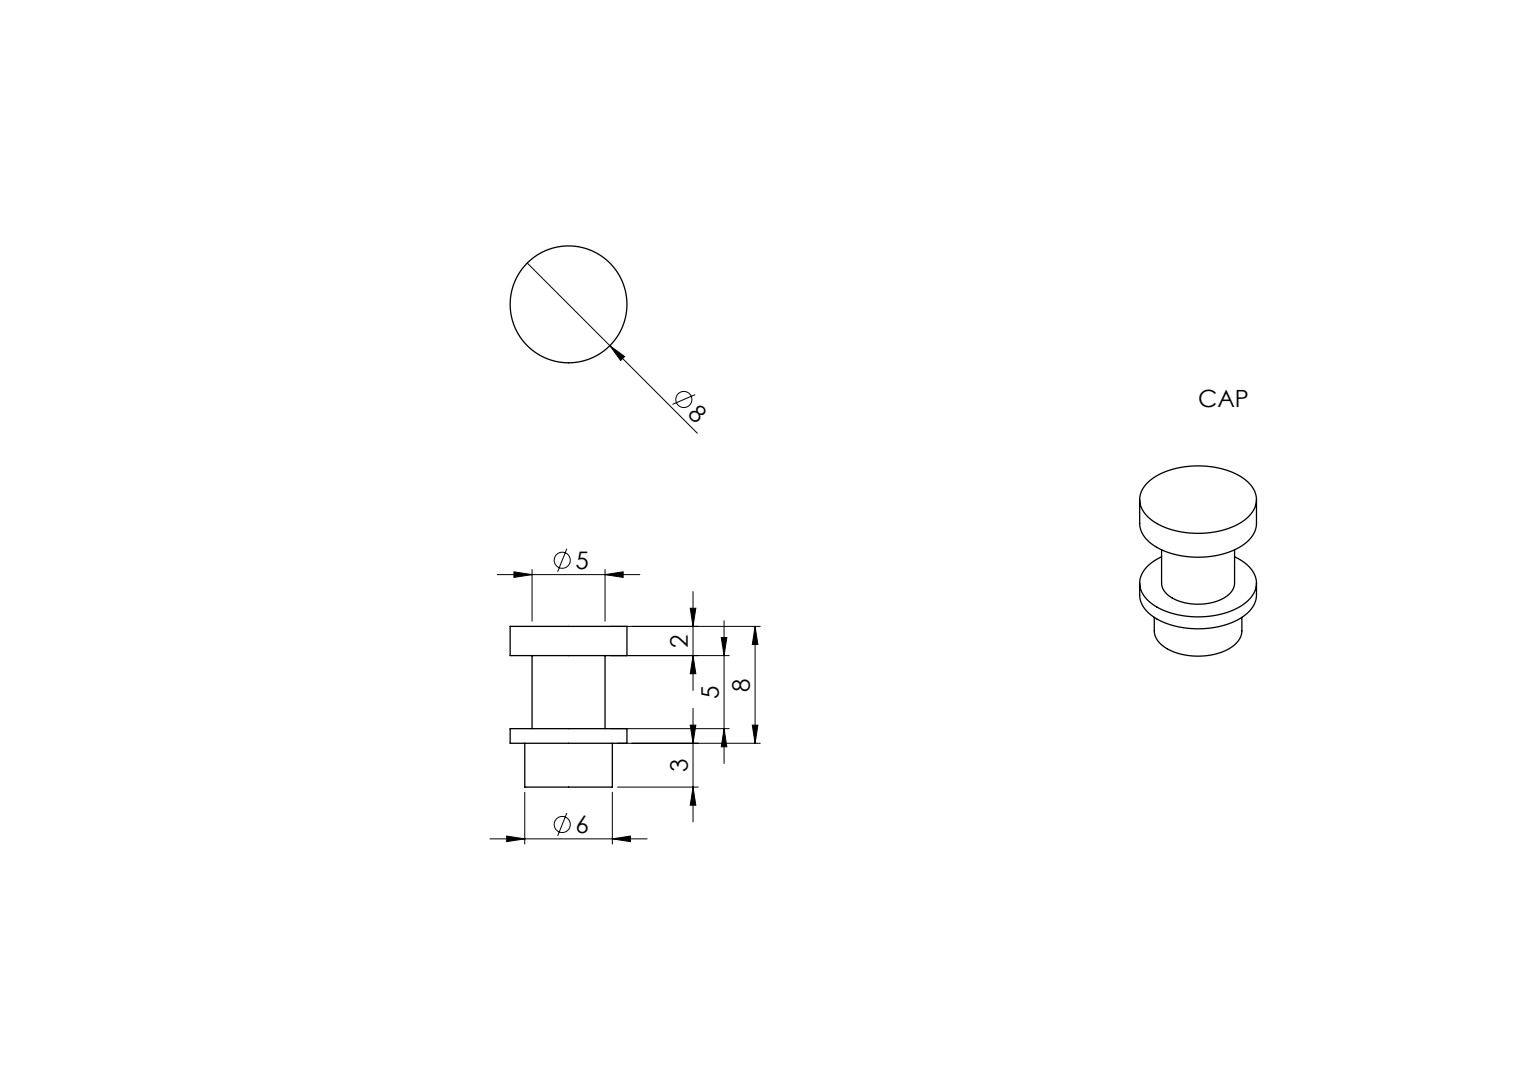
ISO-10303-21;
HEADER;
FILE_DESCRIPTION (('STEP AP214'),
    '1' );
FILE_NAME ('cap.step',
    '2026-10-27T10:49:47',
    ( '' ),
    ( '' ),
    'SwSTEP 2.0',
    'SolidWorks 2026',
    '' );
FILE_SCHEMA (( 'AUTOMOTIVE_DESIGN' ));
ENDSEC;

DATA;
#26=CARTESIAN_POINT ( 'NONE',  ( 4.898587196589412829E-16, 81.00000000000001421, 4.000000000000000000 ) ) ;
#47=( GEOMETRIC_REPRESENTATION_CONTEXT ( 3 ) GLOBAL_UNCERTAINTY_ASSIGNED_CONTEXT ( ( #2399 ) ) GLOBAL_UNIT_ASSIGNED_CONTEXT ( ( #4022, #5674, #2943 ) ) REPRESENTATION_CONTEXT ( 'NONE', 'WORKASPACE' ) );
#72=DIRECTION ( 'NONE',  ( -0.000000000000000000, 1.000000000000000000, -0.000000000000000000 ) ) ;
#89=LINE ( 'NONE', #7305, #4201 ) ;
#131=ADVANCED_FACE ( 'NONE', ( #1342 ), #6353, .T. ) ;
#147=AXIS2_PLACEMENT_3D ( 'NONE', #204, #847, #6661 ) ;
#150=FACE_OUTER_BOUND ( 'NONE', #5421, .T. ) ;
#154=VERTEX_POINT ( 'NONE', #6883 ) ;
#201=VECTOR ( 'NONE', #4183, 1000.000000000000000 ) ;
#204=CARTESIAN_POINT ( 'NONE',  ( 0.000000000000000000, 74.00000000000001421, 0.000000000000000000 ) ) ;
#268=FACE_OUTER_BOUND ( 'NONE', #8425, .T. ) ;
#292=AXIS2_PLACEMENT_3D ( 'NONE', #3378, #6815, #3894 ) ;
#297=DIRECTION ( 'NONE',  ( 0.000000000000000000, 0.000000000000000000, 1.000000000000000000 ) ) ;
#349=PRODUCT_DEFINITION ( 'UNKNOWN', '', #5751, #3204 ) ;
#350=DIRECTION ( 'NONE',  ( 0.000000000000000000, 1.000000000000000000, 0.000000000000000000 ) ) ;
#372=ORIENTED_EDGE ( 'NONE', *, *, #5983, .F. ) ;
#397=CYLINDRICAL_SURFACE ( 'NONE', #2530, 4.000000000000000000 ) ;
#400=EDGE_LOOP ( 'NONE', ( #2352, #922 ) ) ;
#408=ORIENTED_EDGE ( 'NONE', *, *, #9125, .F. ) ;
#409=( GEOMETRIC_REPRESENTATION_CONTEXT ( 3 ) GLOBAL_UNCERTAINTY_ASSIGNED_CONTEXT ( ( #1055 ) ) GLOBAL_UNIT_ASSIGNED_CONTEXT ( ( #5104, #7442, #1066 ) ) REPRESENTATION_CONTEXT ( 'NONE', 'WORKASPACE' ) );
#438=DIRECTION ( 'NONE',  ( -0.000000000000000000, -1.000000000000000000, -0.000000000000000000 ) ) ;
#443=CIRCLE ( 'NONE', #7579, 2.500000000000000000 ) ;
#455=VECTOR ( 'NONE', #7883, 1000.000000000000000 ) ;
#507=CARTESIAN_POINT ( 'NONE',  ( 4.898587196589412829E-16, 73.00000000000001421, 4.000000000000000000 ) ) ;
#537=DIRECTION ( 'NONE',  ( 0.000000000000000000, 0.000000000000000000, 1.000000000000000000 ) ) ;
#582=CARTESIAN_POINT ( 'NONE',  ( 0.000000000000000000, 74.00000000000001421, 2.500000000000000000 ) ) ;
#591=AXIS2_PLACEMENT_3D ( 'NONE', #8216, #7514, #537 ) ;
#594=FACE_OUTER_BOUND ( 'NONE', #5132, .T. ) ;
#612=CIRCLE ( 'NONE', #2974, 3.000000000000000444 ) ;
#624=DIRECTION ( 'NONE',  ( 0.000000000000000000, 0.000000000000000000, -1.000000000000000000 ) ) ;
#634=DIRECTION ( 'NONE',  ( -0.000000000000000000, -1.000000000000000000, -0.000000000000000000 ) ) ;
#641=DIRECTION ( 'NONE',  ( 0.000000000000000000, 1.000000000000000000, 0.000000000000000000 ) ) ;
#690=DIRECTION ( 'NONE',  ( 0.000000000000000000, 0.000000000000000000, 1.000000000000000000 ) ) ;
#691=PRODUCT ( 'cap', 'cap', '', ( #8871 ) ) ;
#724=AXIS2_PLACEMENT_3D ( 'NONE', #8229, #4642, #1153 ) ;
#847=DIRECTION ( 'NONE',  ( 0.000000000000000000, 1.000000000000000000, 0.000000000000000000 ) ) ;
#888=AXIS2_PLACEMENT_3D ( 'NONE', #4026, #9081, #6861 ) ;
#893=CARTESIAN_POINT ( 'NONE',  ( 0.000000000000000000, 79.00000000000001421, 0.000000000000000000 ) ) ;
#922=ORIENTED_EDGE ( 'NONE', *, *, #8343, .T. ) ;
#969=SURFACE_STYLE_USAGE ( .BOTH. , #8693 ) ;
#974=EDGE_LOOP ( 'NONE', ( #8366, #1071 ) ) ;
#989=FACE_BOUND ( 'NONE', #6645, .T. ) ;
#1041=CYLINDRICAL_SURFACE ( 'NONE', #7416, 3.000000000000000444 ) ;
#1048=ORIENTED_EDGE ( 'NONE', *, *, #8424, .T. ) ;
#1055=UNCERTAINTY_MEASURE_WITH_UNIT (LENGTH_MEASURE( 1.000000000000000082E-05 ), #5104, 'distance_accuracy_value', 'NONE');
#1066=( NAMED_UNIT ( * ) SI_UNIT ( $, .STERADIAN. ) SOLID_ANGLE_UNIT ( ) );
#1071=ORIENTED_EDGE ( 'NONE', *, *, #1671, .T. ) ;
#1106=ORIENTED_EDGE ( 'NONE', *, *, #6600, .F. ) ;
#1153=DIRECTION ( 'NONE',  ( 0.000000000000000000, 0.000000000000000000, 1.000000000000000000 ) ) ;
#1168=DIRECTION ( 'NONE',  ( 0.000000000000000000, 0.000000000000000000, 1.000000000000000000 ) ) ;
#1182=CIRCLE ( 'NONE', #724, 3.000000000000000444 ) ;
#1184=EDGE_CURVE ( 'NONE', #3304, #2164, #5654, .T. ) ;
#1191=CIRCLE ( 'NONE', #292, 2.500000000000000000 ) ;
#1216=ORIENTED_EDGE ( 'NONE', *, *, #4101, .T. ) ;
#1230=DIRECTION ( 'NONE',  ( 0.000000000000000000, 0.000000000000000000, 1.000000000000000000 ) ) ;
#1251=AXIS2_PLACEMENT_3D ( 'NONE', #3620, #641, #4139 ) ;
#1330=ORIENTED_EDGE ( 'NONE', *, *, #8424, .F. ) ;
#1333=DIRECTION ( 'NONE',  ( -0.000000000000000000, -1.000000000000000000, -0.000000000000000000 ) ) ;
#1342=FACE_OUTER_BOUND ( 'NONE', #5979, .T. ) ;
#1366=CARTESIAN_POINT ( 'NONE',  ( 0.000000000000000000, 74.00000000000001421, 0.000000000000000000 ) ) ;
#1367=DIRECTION ( 'NONE',  ( 0.000000000000000000, 1.000000000000000000, 0.000000000000000000 ) ) ;
#1372=CARTESIAN_POINT ( 'NONE',  ( 0.000000000000000000, 79.00000000000001421, -4.000000000000000000 ) ) ;
#1423=CARTESIAN_POINT ( 'NONE',  ( 4.898587196589412829E-16, 81.00000000000001421, 4.000000000000000000 ) ) ;
#1434=VERTEX_POINT ( 'NONE', #7055 ) ;
#1465=LINE ( 'NONE', #5884, #5657 ) ;
#1473=CARTESIAN_POINT ( 'NONE',  ( 0.000000000000000000, 81.00000000000001421, 0.000000000000000000 ) ) ;
#1539=CIRCLE ( 'NONE', #1251, 4.000000000000000000 ) ;
#1631=ORIENTED_EDGE ( 'NONE', *, *, #8037, .F. ) ;
#1635=AXIS2_PLACEMENT_3D ( 'NONE', #8434, #6111, #4845 ) ;
#1646=ORIENTED_EDGE ( 'NONE', *, *, #5983, .T. ) ;
#1651=ORIENTED_EDGE ( 'NONE', *, *, #2549, .T. ) ;
#1671=EDGE_CURVE ( 'NONE', #2249, #5349, #3580, .T. ) ;
#1719=PRESENTATION_STYLE_ASSIGNMENT (( #969 ) ) ;
#1822=VERTEX_POINT ( 'NONE', #8975 ) ;
#1853=ORIENTED_EDGE ( 'NONE', *, *, #2021, .F. ) ;
#1854=DIRECTION ( 'NONE',  ( -0.000000000000000000, -1.000000000000000000, -0.000000000000000000 ) ) ;
#1870=SHAPE_DEFINITION_REPRESENTATION ( #2935, #2791 ) ;
#1878=CARTESIAN_POINT ( 'NONE',  ( 0.000000000000000000, 70.00000000000000000, 0.000000000000000000 ) ) ;
#1886=DIRECTION ( 'NONE',  ( 0.000000000000000000, 1.000000000000000000, 0.000000000000000000 ) ) ;
#1892=FACE_OUTER_BOUND ( 'NONE', #5432, .T. ) ;
#1911=ORIENTED_EDGE ( 'NONE', *, *, #6017, .F. ) ;
#1985=ORIENTED_EDGE ( 'NONE', *, *, #8607, .F. ) ;
#2001=CARTESIAN_POINT ( 'NONE',  ( 0.000000000000000000, 81.00000000000001421, 0.000000000000000000 ) ) ;
#2018=EDGE_CURVE ( 'NONE', #3890, #7425, #4835, .T. ) ;
#2021=EDGE_CURVE ( 'NONE', #1822, #7425, #5506, .T. ) ;
#2075=AXIS2_PLACEMENT_3D ( 'NONE', #893, #5822, #7966 ) ;
#2095=AXIS2_PLACEMENT_3D ( 'NONE', #5123, #4435, #8712 ) ;
#2118=AXIS2_PLACEMENT_3D ( 'NONE', #2001, #7761, #2656 ) ;
#2125=DIRECTION ( 'NONE',  ( -0.000000000000000000, -1.000000000000000000, -0.000000000000000000 ) ) ;
#2132=LINE ( 'NONE', #2219, #201 ) ;
#2154=EDGE_CURVE ( 'NONE', #6474, #3890, #612, .T. ) ;
#2164=VERTEX_POINT ( 'NONE', #507 ) ;
#2219=CARTESIAN_POINT ( 'NONE',  ( 0.000000000000000000, 74.00000000000001421, 2.500000000000000000 ) ) ;
#2241=VECTOR ( 'NONE', #72, 1000.000000000000000 ) ;
#2249=VERTEX_POINT ( 'NONE', #9007 ) ;
#2274=CARTESIAN_POINT ( 'NONE',  ( 3.061616997868383141E-16, 79.00000000000001421, -2.500000000000000000 ) ) ;
#2304=EDGE_CURVE ( 'NONE', #6523, #3606, #2746, .T. ) ;
#2352=ORIENTED_EDGE ( 'NONE', *, *, #4698, .T. ) ;
#2392=CARTESIAN_POINT ( 'NONE',  ( 0.000000000000000000, 73.00000000000001421, -4.000000000000000000 ) ) ;
#2399=UNCERTAINTY_MEASURE_WITH_UNIT (LENGTH_MEASURE( 1.000000000000000082E-05 ), #4022, 'distance_accuracy_value', 'NONE');
#2447=FACE_OUTER_BOUND ( 'NONE', #4238, .T. ) ;
#2491=ORIENTED_EDGE ( 'NONE', *, *, #2832, .F. ) ;
#2530=AXIS2_PLACEMENT_3D ( 'NONE', #6216, #1854, #4589 ) ;
#2538=ADVANCED_BREP_SHAPE_REPRESENTATION ( '', ( #5399, #888 ), #7241 ) ;
#2539=CIRCLE ( 'NONE', #7592, 2.500000000000000000 ) ;
#2549=EDGE_CURVE ( 'NONE', #5349, #2876, #1465, .T. ) ;
#2574=ORIENTED_EDGE ( 'NONE', *, *, #3984, .F. ) ;
#2587=MECHANICAL_DESIGN_GEOMETRIC_PRESENTATION_REPRESENTATION('',(#8813),#47);
#2656=DIRECTION ( 'NONE',  ( 0.000000000000000000, 0.000000000000000000, -1.000000000000000000 ) ) ;
#2677=AXIS2_PLACEMENT_3D ( 'NONE', #8411, #634, #5035 ) ;
#2698=DIRECTION ( 'NONE',  ( 0.000000000000000000, 0.000000000000000000, 1.000000000000000000 ) ) ;
#2731=CIRCLE ( 'NONE', #2874, 2.500000000000000000 ) ;
#2746=LINE ( 'NONE', #7895, #2241 ) ;
#2782=ADVANCED_FACE ( 'NONE', ( #8360 ), #397, .T. ) ;
#2791=SHAPE_REPRESENTATION ( 'cap', ( #888 ), #7241 ) ;
#2832=EDGE_CURVE ( 'NONE', #154, #2876, #9188, .T. ) ;
#2874=AXIS2_PLACEMENT_3D ( 'NONE', #6008, #1886, #6200 ) ;
#2876=VERTEX_POINT ( 'NONE', #1372 ) ;
#2907=CYLINDRICAL_SURFACE ( 'NONE', #7179, 2.500000000000000000 ) ;
#2909=FACE_OUTER_BOUND ( 'NONE', #4484, .T. ) ;
#2935=PRODUCT_DEFINITION_SHAPE ( 'NONE', 'NONE',  #349 ) ;
#2943=( NAMED_UNIT ( * ) SI_UNIT ( $, .STERADIAN. ) SOLID_ANGLE_UNIT ( ) );
#2952=DIRECTION ( 'NONE',  ( 0.000000000000000000, 1.000000000000000000, 0.000000000000000000 ) ) ;
#2974=AXIS2_PLACEMENT_3D ( 'NONE', #8866, #9054, #2698 ) ;
#2977=CIRCLE ( 'NONE', #3717, 3.000000000000000444 ) ;
#2998=CARTESIAN_POINT ( 'NONE',  ( 3.673940397442060361E-16, 73.00000000000001421, 3.000000000000000444 ) ) ;
#3039=DIRECTION ( 'NONE',  ( -0.000000000000000000, -1.000000000000000000, -0.000000000000000000 ) ) ;
#3043=CIRCLE ( 'NONE', #8238, 4.000000000000000000 ) ;
#3047=CARTESIAN_POINT ( 'NONE',  ( 0.000000000000000000, 73.00000000000001421, 0.000000000000000000 ) ) ;
#3055=PLANE ( 'NONE',  #147 ) ;
#3077=FILL_AREA_STYLE ('',( #8043 ) ) ;
#3084=EDGE_LOOP ( 'NONE', ( #7913, #1646 ) ) ;
#3121=PLANE ( 'NONE',  #1635 ) ;
#3133=AXIS2_PLACEMENT_3D ( 'NONE', #3047, #3741, #8659 ) ;
#3135=EDGE_CURVE ( 'NONE', #6474, #1822, #5027, .T. ) ;
#3155=ORIENTED_EDGE ( 'NONE', *, *, #1671, .F. ) ;
#3163=ADVANCED_FACE ( 'NONE', ( #989, #5222 ), #3055, .T. ) ;
#3167=CARTESIAN_POINT ( 'NONE',  ( 0.000000000000000000, 74.00000000000001421, 0.000000000000000000 ) ) ;
#3204=PRODUCT_DEFINITION_CONTEXT ( 'detailed design', #5531, 'design' ) ;
#3205=VERTEX_POINT ( 'NONE', #2392 ) ;
#3237=CYLINDRICAL_SURFACE ( 'NONE', #7792, 4.000000000000000000 ) ;
#3256=ORIENTED_EDGE ( 'NONE', *, *, #3453, .T. ) ;
#3288=DIRECTION ( 'NONE',  ( 0.000000000000000000, 0.000000000000000000, 1.000000000000000000 ) ) ;
#3304=VERTEX_POINT ( 'NONE', #6759 ) ;
#3314=DIRECTION ( 'NONE',  ( -0.000000000000000000, -1.000000000000000000, -0.000000000000000000 ) ) ;
#3321=ORIENTED_EDGE ( 'NONE', *, *, #8037, .T. ) ;
#3378=CARTESIAN_POINT ( 'NONE',  ( 0.000000000000000000, 79.00000000000001421, 0.000000000000000000 ) ) ;
#3453=EDGE_CURVE ( 'NONE', #4194, #6523, #2539, .T. ) ;
#3580=CIRCLE ( 'NONE', #2095, 4.000000000000000000 ) ;
#3606=VERTEX_POINT ( 'NONE', #2274 ) ;
#3620=CARTESIAN_POINT ( 'NONE',  ( 0.000000000000000000, 74.00000000000001421, 0.000000000000000000 ) ) ;
#3643=CARTESIAN_POINT ( 'NONE',  ( 0.000000000000000000, 70.00000000000000000, 0.000000000000000000 ) ) ;
#3655=ORIENTED_EDGE ( 'NONE', *, *, #8343, .F. ) ;
#3717=AXIS2_PLACEMENT_3D ( 'NONE', #4887, #4762, #1230 ) ;
#3741=DIRECTION ( 'NONE',  ( 0.000000000000000000, 1.000000000000000000, 0.000000000000000000 ) ) ;
#3743=FACE_OUTER_BOUND ( 'NONE', #6302, .T. ) ;
#3772=SURFACE_STYLE_FILL_AREA ( #3077 ) ;
#3777=ORIENTED_EDGE ( 'NONE', *, *, #9125, .T. ) ;
#3794=CARTESIAN_POINT ( 'NONE',  ( 0.000000000000000000, 73.00000000000001421, -3.000000000000000444 ) ) ;
#3847=DIRECTION ( 'NONE',  ( -0.000000000000000000, -1.000000000000000000, -0.000000000000000000 ) ) ;
#3868=CIRCLE ( 'NONE', #5934, 4.000000000000000000 ) ;
#3890=VERTEX_POINT ( 'NONE', #2998 ) ;
#3894=DIRECTION ( 'NONE',  ( 0.000000000000000000, 0.000000000000000000, 1.000000000000000000 ) ) ;
#3900=ORIENTED_EDGE ( 'NONE', *, *, #1184, .T. ) ;
#3903=CARTESIAN_POINT ( 'NONE',  ( 3.673940397442060361E-16, 70.00000000000000000, 3.000000000000000444 ) ) ;
#3935=CARTESIAN_POINT ( 'NONE',  ( 0.000000000000000000, 73.00000000000001421, -3.000000000000000444 ) ) ;
#3984=EDGE_CURVE ( 'NONE', #2164, #3205, #7138, .T. ) ;
#4022=( LENGTH_UNIT ( ) NAMED_UNIT ( * ) SI_UNIT ( .MILLI., .METRE. ) );
#4026=CARTESIAN_POINT ( 'NONE',  ( 0.000000000000000000, 0.000000000000000000, 0.000000000000000000 ) ) ;
#4101=EDGE_CURVE ( 'NONE', #5172, #3205, #89, .T. ) ;
#4118=DIRECTION ( 'NONE',  ( -0.000000000000000000, -1.000000000000000000, -0.000000000000000000 ) ) ;
#4139=DIRECTION ( 'NONE',  ( 0.000000000000000000, 0.000000000000000000, 1.000000000000000000 ) ) ;
#4183=DIRECTION ( 'NONE',  ( -0.000000000000000000, 1.000000000000000000, -0.000000000000000000 ) ) ;
#4194=VERTEX_POINT ( 'NONE', #582 ) ;
#4201=VECTOR ( 'NONE', #3039, 1000.000000000000000 ) ;
#4238=EDGE_LOOP ( 'NONE', ( #1631, #1106, #1651, #5055 ) ) ;
#4275=ADVANCED_FACE ( 'NONE', ( #2909 ), #5683, .T. ) ;
#4316=DIRECTION ( 'NONE',  ( 0.000000000000000000, 1.000000000000000000, 0.000000000000000000 ) ) ;
#4349=EDGE_LOOP ( 'NONE', ( #6694, #6748 ) ) ;
#4435=DIRECTION ( 'NONE',  ( 0.000000000000000000, 1.000000000000000000, 0.000000000000000000 ) ) ;
#4466=ORIENTED_EDGE ( 'NONE', *, *, #3453, .F. ) ;
#4484=EDGE_LOOP ( 'NONE', ( #6407, #6798, #7135, #4561 ) ) ;
#4561=ORIENTED_EDGE ( 'NONE', *, *, #2021, .T. ) ;
#4589=DIRECTION ( 'NONE',  ( 0.000000000000000000, 0.000000000000000000, -1.000000000000000000 ) ) ;
#4592=ORIENTED_EDGE ( 'NONE', *, *, #2304, .F. ) ;
#4627=DIRECTION ( 'NONE',  ( 0.000000000000000000, 0.000000000000000000, -1.000000000000000000 ) ) ;
#4631=DIRECTION ( 'NONE',  ( 0.000000000000000000, 1.000000000000000000, 0.000000000000000000 ) ) ;
#4642=DIRECTION ( 'NONE',  ( 0.000000000000000000, 1.000000000000000000, 0.000000000000000000 ) ) ;
#4674=DIRECTION ( 'NONE',  ( -0.000000000000000000, -1.000000000000000000, -0.000000000000000000 ) ) ;
#4698=EDGE_CURVE ( 'NONE', #1434, #3606, #2731, .T. ) ;
#4762=DIRECTION ( 'NONE',  ( 0.000000000000000000, 1.000000000000000000, 0.000000000000000000 ) ) ;
#4835=LINE ( 'NONE', #8244, #7738 ) ;
#4845=DIRECTION ( 'NONE',  ( 0.000000000000000000, -0.000000000000000000, 1.000000000000000000 ) ) ;
#4887=CARTESIAN_POINT ( 'NONE',  ( 0.000000000000000000, 70.00000000000000000, 0.000000000000000000 ) ) ;
#4892=DIRECTION ( 'NONE',  ( -0.000000000000000000, 1.000000000000000000, -0.000000000000000000 ) ) ;
#4962=CARTESIAN_POINT ( 'NONE',  ( 0.000000000000000000, 74.00000000000001421, 0.000000000000000000 ) ) ;
#4995=FACE_OUTER_BOUND ( 'NONE', #974, .T. ) ;
#5010=EDGE_LOOP ( 'NONE', ( #4592, #8857, #9090, #3655 ) ) ;
#5016=ADVANCED_FACE ( 'NONE', ( #5638 ), #2907, .T. ) ;
#5027=LINE ( 'NONE', #3794, #455 ) ;
#5035=DIRECTION ( 'NONE',  ( 0.000000000000000000, 0.000000000000000000, -1.000000000000000000 ) ) ;
#5053=DIRECTION ( 'NONE',  ( 0.000000000000000000, 1.000000000000000000, 0.000000000000000000 ) ) ;
#5055=ORIENTED_EDGE ( 'NONE', *, *, #8607, .T. ) ;
#5104=( LENGTH_UNIT ( ) NAMED_UNIT ( * ) SI_UNIT ( .MILLI., .METRE. ) );
#5110=ORIENTED_EDGE ( 'NONE', *, *, #4698, .F. ) ;
#5123=CARTESIAN_POINT ( 'NONE',  ( 0.000000000000000000, 81.00000000000001421, 0.000000000000000000 ) ) ;
#5132=EDGE_LOOP ( 'NONE', ( #372, #3900, #8266, #7731 ) ) ;
#5172=VERTEX_POINT ( 'NONE', #7412 ) ;
#5222=FACE_OUTER_BOUND ( 'NONE', #3084, .T. ) ;
#5314=DIRECTION ( 'NONE',  ( 0.000000000000000000, 1.000000000000000000, 0.000000000000000000 ) ) ;
#5349=VERTEX_POINT ( 'NONE', #5358 ) ;
#5358=CARTESIAN_POINT ( 'NONE',  ( 0.000000000000000000, 81.00000000000001421, -4.000000000000000000 ) ) ;
#5399=MANIFOLD_SOLID_BREP ( 'Cut-Extrude-Thin1', #6088 ) ;
#5421=EDGE_LOOP ( 'NONE', ( #1985, #2491 ) ) ;
#5432=EDGE_LOOP ( 'NONE', ( #8598, #6476, #3777, #8148 ) ) ;
#5506=CIRCLE ( 'NONE', #6100, 3.000000000000000444 ) ;
#5531=APPLICATION_CONTEXT ( 'automotive_design' ) ;
#5608=COLOUR_RGB ( '',0.8941176470588234615, 0.8941176470588234615, 0.8941176470588234615 ) ;
#5638=FACE_OUTER_BOUND ( 'NONE', #5010, .T. ) ;
#5654=LINE ( 'NONE', #1423, #6148 ) ;
#5657=VECTOR ( 'NONE', #3847, 1000.000000000000000 ) ;
#5674=( NAMED_UNIT ( * ) PLANE_ANGLE_UNIT ( ) SI_UNIT ( $, .RADIAN. ) );
#5683=CYLINDRICAL_SURFACE ( 'NONE', #7768, 3.000000000000000444 ) ;
#5751=PRODUCT_DEFINITION_FORMATION_WITH_SPECIFIED_SOURCE ( 'ANY', '', #691, .NOT_KNOWN. ) ;
#5782=AXIS2_PLACEMENT_3D ( 'NONE', #7174, #6466, #8059 ) ;
#5787=EDGE_LOOP ( 'NONE', ( #6426, #7090, #1216, #1048 ) ) ;
#5822=DIRECTION ( 'NONE',  ( 0.000000000000000000, 1.000000000000000000, 0.000000000000000000 ) ) ;
#5884=CARTESIAN_POINT ( 'NONE',  ( 0.000000000000000000, 81.00000000000001421, -4.000000000000000000 ) ) ;
#5914=PLANE ( 'NONE',  #7123 ) ;
#5934=AXIS2_PLACEMENT_3D ( 'NONE', #8855, #4631, #3288 ) ;
#5979=EDGE_LOOP ( 'NONE', ( #3155, #3321, #6412, #7752 ) ) ;
#5983=EDGE_CURVE ( 'NONE', #3304, #5172, #1539, .T. ) ;
#6008=CARTESIAN_POINT ( 'NONE',  ( 0.000000000000000000, 79.00000000000001421, 0.000000000000000000 ) ) ;
#6017=EDGE_CURVE ( 'NONE', #4194, #1434, #2132, .T. ) ;
#6061=CARTESIAN_POINT ( 'NONE',  ( 3.061616997868383141E-16, 74.00000000000001421, -2.500000000000000000 ) ) ;
#6068=CARTESIAN_POINT ( 'NONE',  ( 0.000000000000000000, 79.00000000000001421, 0.000000000000000000 ) ) ;
#6084=ADVANCED_FACE ( 'NONE', ( #4995 ), #6400, .T. ) ;
#6088=CLOSED_SHELL ( 'NONE', ( #131, #8881, #6622, #7934, #2782, #4275, #8600, #9033, #3163, #8563, #5016, #6084, #6475 ) ) ;
#6100=AXIS2_PLACEMENT_3D ( 'NONE', #1878, #7541, #1168 ) ;
#6111=DIRECTION ( 'NONE',  ( 0.000000000000000000, 1.000000000000000000, 0.000000000000000000 ) ) ;
#6148=VECTOR ( 'NONE', #2125, 1000.000000000000000 ) ;
#6163=CARTESIAN_POINT ( 'NONE',  ( 0.000000000000000000, 73.00000000000001421, 0.000000000000000000 ) ) ;
#6200=DIRECTION ( 'NONE',  ( 0.000000000000000000, 0.000000000000000000, 1.000000000000000000 ) ) ;
#6216=CARTESIAN_POINT ( 'NONE',  ( 0.000000000000000000, 81.00000000000001421, 0.000000000000000000 ) ) ;
#6302=EDGE_LOOP ( 'NONE', ( #1853, #408 ) ) ;
#6321=EDGE_LOOP ( 'NONE', ( #3256, #9044, #5110, #1911 ) ) ;
#6353=CYLINDRICAL_SURFACE ( 'NONE', #2118, 4.000000000000000000 ) ;
#6400=PLANE ( 'NONE',  #8231 ) ;
#6407=ORIENTED_EDGE ( 'NONE', *, *, #2018, .F. ) ;
#6412=ORIENTED_EDGE ( 'NONE', *, *, #2832, .T. ) ;
#6426=ORIENTED_EDGE ( 'NONE', *, *, #1184, .F. ) ;
#6444=DIRECTION ( 'NONE',  ( 0.000000000000000000, -0.000000000000000000, 1.000000000000000000 ) ) ;
#6466=DIRECTION ( 'NONE',  ( 0.000000000000000000, 1.000000000000000000, 0.000000000000000000 ) ) ;
#6474=VERTEX_POINT ( 'NONE', #3935 ) ;
#6475=ADVANCED_FACE ( 'NONE', ( #2447 ), #3237, .T. ) ;
#6476=ORIENTED_EDGE ( 'NONE', *, *, #2018, .T. ) ;
#6513=DIRECTION ( 'NONE',  ( 0.000000000000000000, -0.000000000000000000, 1.000000000000000000 ) ) ;
#6523=VERTEX_POINT ( 'NONE', #6061 ) ;
#6600=EDGE_CURVE ( 'NONE', #5349, #2249, #3043, .T. ) ;
#6622=ADVANCED_FACE ( 'NONE', ( #1892 ), #1041, .T. ) ;
#6639=FACE_BOUND ( 'NONE', #4349, .T. ) ;
#6645=EDGE_LOOP ( 'NONE', ( #4466, #8198 ) ) ;
#6661=DIRECTION ( 'NONE',  ( 0.000000000000000000, -0.000000000000000000, 1.000000000000000000 ) ) ;
#6694=ORIENTED_EDGE ( 'NONE', *, *, #2154, .T. ) ;
#6748=ORIENTED_EDGE ( 'NONE', *, *, #7785, .T. ) ;
#6759=CARTESIAN_POINT ( 'NONE',  ( 4.898587196589412829E-16, 74.00000000000001421, 4.000000000000000000 ) ) ;
#6798=ORIENTED_EDGE ( 'NONE', *, *, #2154, .F. ) ;
#6804=MECHANICAL_DESIGN_GEOMETRIC_PRESENTATION_REPRESENTATION('',(#7692),#409);
#6815=DIRECTION ( 'NONE',  ( 0.000000000000000000, 1.000000000000000000, 0.000000000000000000 ) ) ;
#6832=CIRCLE ( 'NONE', #5782, 4.000000000000000000 ) ;
#6861=DIRECTION ( 'NONE',  ( 1.000000000000000000, 0.000000000000000000, 0.000000000000000000 ) ) ;
#6883=CARTESIAN_POINT ( 'NONE',  ( 4.898587196589412829E-16, 79.00000000000001421, 4.000000000000000000 ) ) ;
#6997=DIRECTION ( 'NONE',  ( 0.000000000000000000, 0.000000000000000000, 1.000000000000000000 ) ) ;
#7055=CARTESIAN_POINT ( 'NONE',  ( 0.000000000000000000, 79.00000000000001421, 2.500000000000000000 ) ) ;
#7090=ORIENTED_EDGE ( 'NONE', *, *, #8447, .F. ) ;
#7123=AXIS2_PLACEMENT_3D ( 'NONE', #3643, #2952, #6513 ) ;
#7135=ORIENTED_EDGE ( 'NONE', *, *, #3135, .T. ) ;
#7138=CIRCLE ( 'NONE', #3133, 4.000000000000000000 ) ;
#7173=DIRECTION ( 'NONE',  ( 0.000000000000000000, 0.000000000000000000, 1.000000000000000000 ) ) ;
#7174=CARTESIAN_POINT ( 'NONE',  ( 0.000000000000000000, 79.00000000000001421, 0.000000000000000000 ) ) ;
#7179=AXIS2_PLACEMENT_3D ( 'NONE', #1366, #4892, #7173 ) ;
#7241=( GEOMETRIC_REPRESENTATION_CONTEXT ( 3 ) GLOBAL_UNCERTAINTY_ASSIGNED_CONTEXT ( ( #7475 ) ) GLOBAL_UNIT_ASSIGNED_CONTEXT ( ( #7774, #9155, #8426 ) ) REPRESENTATION_CONTEXT ( 'NONE', 'WORKASPACE' ) );
#7247=FACE_OUTER_BOUND ( 'NONE', #6321, .T. ) ;
#7305=CARTESIAN_POINT ( 'NONE',  ( 0.000000000000000000, 81.00000000000001421, -4.000000000000000000 ) ) ;
#7412=CARTESIAN_POINT ( 'NONE',  ( 0.000000000000000000, 74.00000000000001421, -4.000000000000000000 ) ) ;
#7416=AXIS2_PLACEMENT_3D ( 'NONE', #6163, #4674, #8167 ) ;
#7419=CARTESIAN_POINT ( 'NONE',  ( 0.000000000000000000, 81.00000000000001421, 0.000000000000000000 ) ) ;
#7425=VERTEX_POINT ( 'NONE', #3903 ) ;
#7442=( NAMED_UNIT ( * ) PLANE_ANGLE_UNIT ( ) SI_UNIT ( $, .RADIAN. ) );
#7475=UNCERTAINTY_MEASURE_WITH_UNIT (LENGTH_MEASURE( 1.000000000000000082E-05 ), #7774, 'distance_accuracy_value', 'NONE');
#7514=DIRECTION ( 'NONE',  ( 0.000000000000000000, 1.000000000000000000, 0.000000000000000000 ) ) ;
#7541=DIRECTION ( 'NONE',  ( 0.000000000000000000, 1.000000000000000000, 0.000000000000000000 ) ) ;
#7579=AXIS2_PLACEMENT_3D ( 'NONE', #7744, #1367, #6997 ) ;
#7583=AXIS2_PLACEMENT_3D ( 'NONE', #6068, #350, #8904 ) ;
#7592=AXIS2_PLACEMENT_3D ( 'NONE', #4962, #5053, #690 ) ;
#7692=STYLED_ITEM ( 'NONE', ( #1719 ), #2538 ) ;
#7708=LINE ( 'NONE', #26, #9049 ) ;
#7723=CIRCLE ( 'NONE', #591, 4.000000000000000000 ) ;
#7731=ORIENTED_EDGE ( 'NONE', *, *, #4101, .F. ) ;
#7738=VECTOR ( 'NONE', #3314, 1000.000000000000000 ) ;
#7744=CARTESIAN_POINT ( 'NONE',  ( 0.000000000000000000, 74.00000000000001421, 0.000000000000000000 ) ) ;
#7752=ORIENTED_EDGE ( 'NONE', *, *, #2549, .F. ) ;
#7761=DIRECTION ( 'NONE',  ( -0.000000000000000000, -1.000000000000000000, -0.000000000000000000 ) ) ;
#7768=AXIS2_PLACEMENT_3D ( 'NONE', #8440, #4118, #624 ) ;
#7774=( LENGTH_UNIT ( ) NAMED_UNIT ( * ) SI_UNIT ( .MILLI., .METRE. ) );
#7785=EDGE_CURVE ( 'NONE', #3890, #6474, #1182, .T. ) ;
#7792=AXIS2_PLACEMENT_3D ( 'NONE', #7419, #438, #4627 ) ;
#7883=DIRECTION ( 'NONE',  ( -0.000000000000000000, -1.000000000000000000, -0.000000000000000000 ) ) ;
#7895=CARTESIAN_POINT ( 'NONE',  ( 3.061616997868383141E-16, 74.00000000000001421, -2.500000000000000000 ) ) ;
#7913=ORIENTED_EDGE ( 'NONE', *, *, #8447, .T. ) ;
#7934=ADVANCED_FACE ( 'NONE', ( #594 ), #9142, .T. ) ;
#7951=CYLINDRICAL_SURFACE ( 'NONE', #8171, 2.500000000000000000 ) ;
#7965=APPLICATION_CONTEXT ( 'automotive_design' ) ;
#7966=DIRECTION ( 'NONE',  ( 0.000000000000000000, -0.000000000000000000, 1.000000000000000000 ) ) ;
#8010=PLANE ( 'NONE',  #2075 ) ;
#8037=EDGE_CURVE ( 'NONE', #2249, #154, #7708, .T. ) ;
#8042=DIRECTION ( 'NONE',  ( -0.000000000000000000, 1.000000000000000000, -0.000000000000000000 ) ) ;
#8043=FILL_AREA_STYLE_COLOUR ( '', #5608 ) ;
#8059=DIRECTION ( 'NONE',  ( 0.000000000000000000, 0.000000000000000000, 1.000000000000000000 ) ) ;
#8148=ORIENTED_EDGE ( 'NONE', *, *, #3135, .F. ) ;
#8167=DIRECTION ( 'NONE',  ( 0.000000000000000000, 0.000000000000000000, -1.000000000000000000 ) ) ;
#8171=AXIS2_PLACEMENT_3D ( 'NONE', #3167, #8042, #8785 ) ;
#8198=ORIENTED_EDGE ( 'NONE', *, *, #8471, .F. ) ;
#8216=CARTESIAN_POINT ( 'NONE',  ( 0.000000000000000000, 73.00000000000001421, 0.000000000000000000 ) ) ;
#8229=CARTESIAN_POINT ( 'NONE',  ( 0.000000000000000000, 73.00000000000001421, 0.000000000000000000 ) ) ;
#8231=AXIS2_PLACEMENT_3D ( 'NONE', #1473, #4316, #6444 ) ;
#8238=AXIS2_PLACEMENT_3D ( 'NONE', #8989, #5314, #297 ) ;
#8244=CARTESIAN_POINT ( 'NONE',  ( 3.673940397442060361E-16, 73.00000000000001421, 3.000000000000000444 ) ) ;
#8266=ORIENTED_EDGE ( 'NONE', *, *, #3984, .T. ) ;
#8343=EDGE_CURVE ( 'NONE', #3606, #1434, #1191, .T. ) ;
#8360=FACE_OUTER_BOUND ( 'NONE', #5787, .T. ) ;
#8366=ORIENTED_EDGE ( 'NONE', *, *, #6600, .T. ) ;
#8411=CARTESIAN_POINT ( 'NONE',  ( 0.000000000000000000, 81.00000000000001421, 0.000000000000000000 ) ) ;
#8424=EDGE_CURVE ( 'NONE', #3205, #2164, #7723, .T. ) ;
#8425=EDGE_LOOP ( 'NONE', ( #1330, #2574 ) ) ;
#8426=( NAMED_UNIT ( * ) SI_UNIT ( $, .STERADIAN. ) SOLID_ANGLE_UNIT ( ) );
#8434=CARTESIAN_POINT ( 'NONE',  ( 0.000000000000000000, 73.00000000000001421, 0.000000000000000000 ) ) ;
#8440=CARTESIAN_POINT ( 'NONE',  ( 0.000000000000000000, 73.00000000000001421, 0.000000000000000000 ) ) ;
#8447=EDGE_CURVE ( 'NONE', #5172, #3304, #3868, .T. ) ;
#8471=EDGE_CURVE ( 'NONE', #6523, #4194, #443, .T. ) ;
#8563=ADVANCED_FACE ( 'NONE', ( #8569, #150 ), #8010, .F. ) ;
#8569=FACE_BOUND ( 'NONE', #400, .T. ) ;
#8598=ORIENTED_EDGE ( 'NONE', *, *, #7785, .F. ) ;
#8600=ADVANCED_FACE ( 'NONE', ( #3743 ), #5914, .F. ) ;
#8607=EDGE_CURVE ( 'NONE', #2876, #154, #6832, .T. ) ;
#8659=DIRECTION ( 'NONE',  ( 0.000000000000000000, 0.000000000000000000, 1.000000000000000000 ) ) ;
#8693=SURFACE_SIDE_STYLE ('',( #3772 ) ) ;
#8712=DIRECTION ( 'NONE',  ( 0.000000000000000000, 0.000000000000000000, 1.000000000000000000 ) ) ;
#8738=SHAPE_REPRESENTATION_RELATIONSHIP ( 'NONE' , 'NONE' ,  #2791, #2538 ) ;
#8785=DIRECTION ( 'NONE',  ( 0.000000000000000000, 0.000000000000000000, 1.000000000000000000 ) ) ;
#8813=STYLED_ITEM('',(#9218),#5399);
#8855=CARTESIAN_POINT ( 'NONE',  ( 0.000000000000000000, 74.00000000000001421, 0.000000000000000000 ) ) ;
#8857=ORIENTED_EDGE ( 'NONE', *, *, #8471, .T. ) ;
#8866=CARTESIAN_POINT ( 'NONE',  ( 0.000000000000000000, 73.00000000000001421, 0.000000000000000000 ) ) ;
#8871=PRODUCT_CONTEXT ( 'NONE', #7965, 'mechanical' ) ;
#8881=ADVANCED_FACE ( 'NONE', ( #7247 ), #7951, .T. ) ;
#8904=DIRECTION ( 'NONE',  ( 0.000000000000000000, 0.000000000000000000, 1.000000000000000000 ) ) ;
#8975=CARTESIAN_POINT ( 'NONE',  ( 0.000000000000000000, 70.00000000000000000, -3.000000000000000444 ) ) ;
#8989=CARTESIAN_POINT ( 'NONE',  ( 0.000000000000000000, 81.00000000000001421, 0.000000000000000000 ) ) ;
#9007=CARTESIAN_POINT ( 'NONE',  ( 4.898587196589412829E-16, 81.00000000000001421, 4.000000000000000000 ) ) ;
#9033=ADVANCED_FACE ( 'NONE', ( #6639, #268 ), #3121, .F. ) ;
#9044=ORIENTED_EDGE ( 'NONE', *, *, #2304, .T. ) ;
#9049=VECTOR ( 'NONE', #1333, 1000.000000000000000 ) ;
#9054=DIRECTION ( 'NONE',  ( 0.000000000000000000, 1.000000000000000000, 0.000000000000000000 ) ) ;
#9081=DIRECTION ( 'NONE',  ( 0.000000000000000000, 0.000000000000000000, 1.000000000000000000 ) ) ;
#9090=ORIENTED_EDGE ( 'NONE', *, *, #6017, .T. ) ;
#9125=EDGE_CURVE ( 'NONE', #7425, #1822, #2977, .T. ) ;
#9142=CYLINDRICAL_SURFACE ( 'NONE', #2677, 4.000000000000000000 ) ;
#9155=( NAMED_UNIT ( * ) PLANE_ANGLE_UNIT ( ) SI_UNIT ( $, .RADIAN. ) );
#9188=CIRCLE ( 'NONE', #7583, 4.000000000000000000 ) ;
#9212=COLOUR_RGB('Sky Blue',0.24,0.69,0.87);
#9213=FILL_AREA_STYLE_COLOUR('',#9212);
#9214=FILL_AREA_STYLE('',(#9213));
#9215=SURFACE_STYLE_FILL_AREA(#9214);
#9216=SURFACE_SIDE_STYLE('',(#9215));
#9217=SURFACE_STYLE_USAGE(.BOTH.,#9216);
#9218=PRESENTATION_STYLE_ASSIGNMENT((#9217));
ENDSEC;
END-ISO-10303-21;
